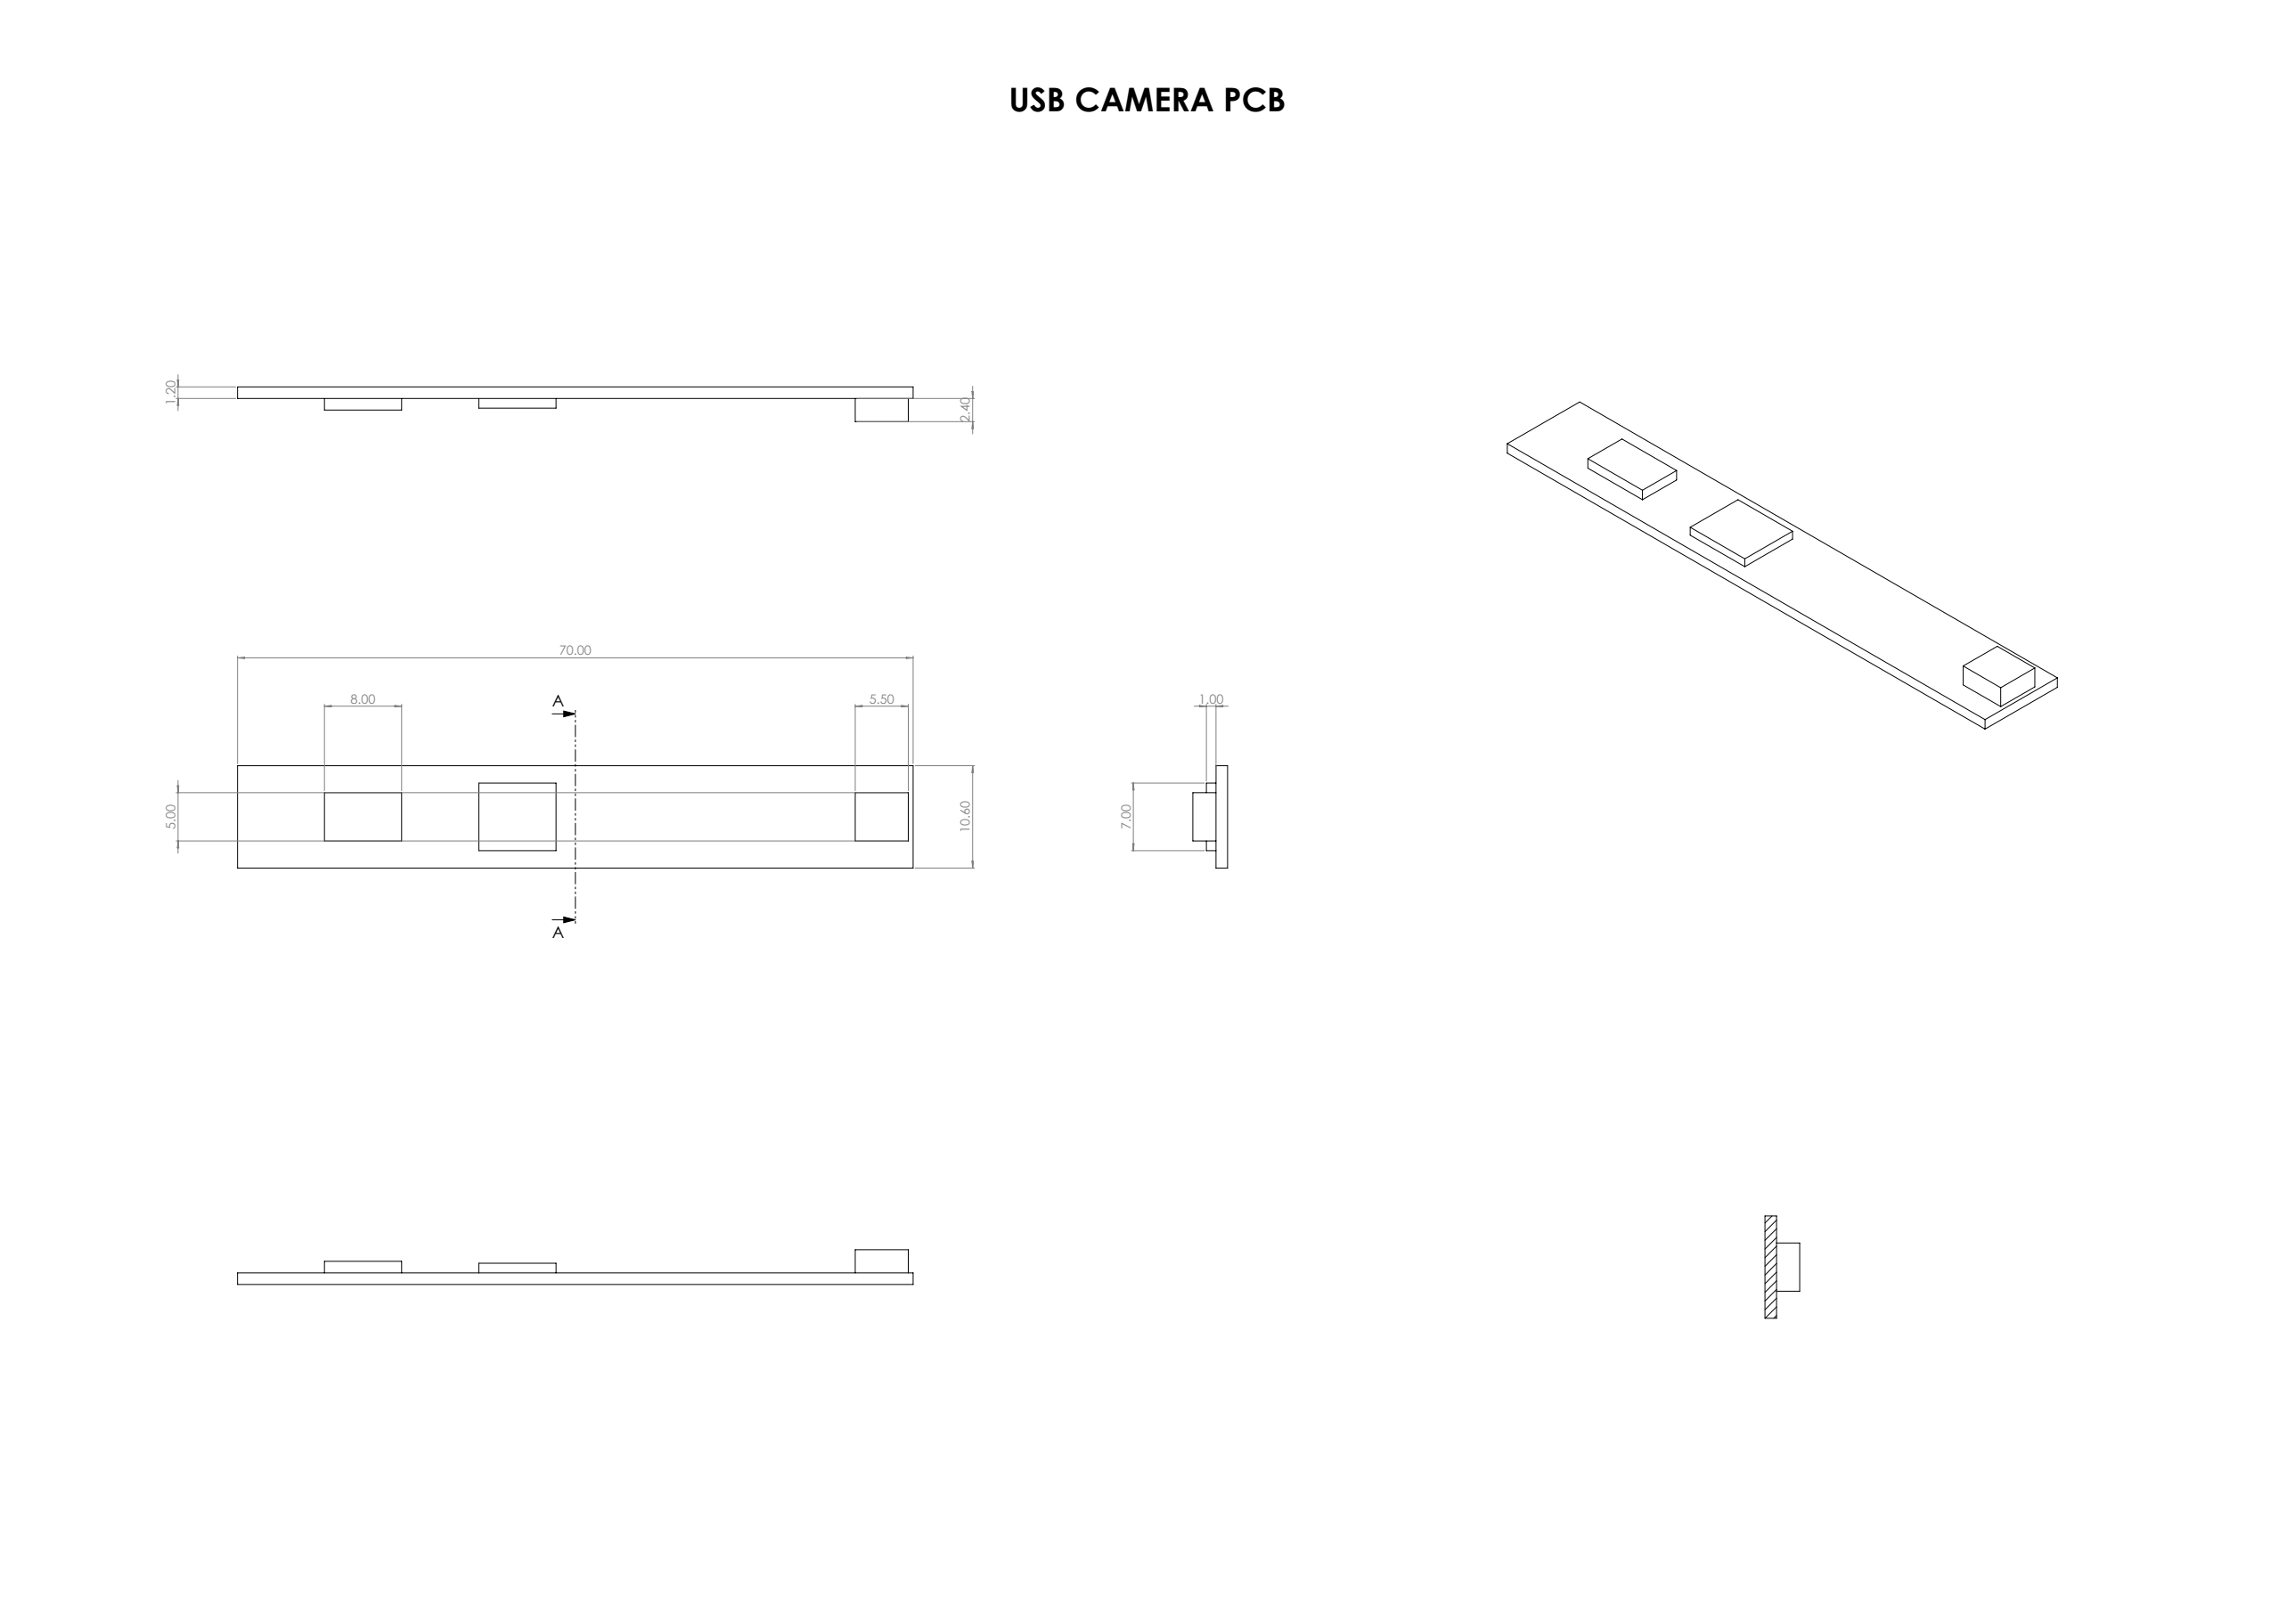
ISO-10303-21;
HEADER;
/* Generated by software containing ST-Developer
 * from STEP Tools, Inc. (www.steptools.com) 
 */

FILE_DESCRIPTION(
/* description */ (''),
/* implementation_level */ '2;1');

FILE_NAME(
/* name */ '05_USB_Camera_PCB.step',
/* time_stamp */ '2026-10-21T02:01:14-07:00',
/* author */ (''),
/* organization */ (''),
/* preprocessor_version */ 'ST-DEVELOPER v20.2',
/* originating_system */ 'Autodesk Translation Framework v15.15.0.0',
/* authorisation */ '');

FILE_SCHEMA (('AUTOMOTIVE_DESIGN { 1 0 10303 214 3 1 1 }'));
ENDSEC;

DATA;
#10=MECHANICAL_DESIGN_GEOMETRIC_PRESENTATION_REPRESENTATION('',(#618),#37181);
#592=SHAPE_REPRESENTATION_RELATIONSHIP('SRR','None',#37242,#605);
#605=ADVANCED_BREP_SHAPE_REPRESENTATION('',(#631),#37172);
#618=STYLED_ITEM('',(#37387),#631);
#631=MANIFOLD_SOLID_BREP('Body1',#14780);
#671=FACE_BOUND('',#2587,.T.);
#672=FACE_BOUND('',#2588,.T.);
#673=FACE_BOUND('',#2589,.T.);
#1696=FACE_OUTER_BOUND('',#2567,.T.);
#1697=FACE_OUTER_BOUND('',#2568,.T.);
#1698=FACE_OUTER_BOUND('',#2569,.T.);
#1699=FACE_OUTER_BOUND('',#2570,.T.);
#1700=FACE_OUTER_BOUND('',#2571,.T.);
#1701=FACE_OUTER_BOUND('',#2572,.T.);
#1702=FACE_OUTER_BOUND('',#2573,.T.);
#1703=FACE_OUTER_BOUND('',#2574,.T.);
#1704=FACE_OUTER_BOUND('',#2575,.T.);
#1705=FACE_OUTER_BOUND('',#2576,.T.);
#1706=FACE_OUTER_BOUND('',#2577,.T.);
#1707=FACE_OUTER_BOUND('',#2578,.T.);
#1708=FACE_OUTER_BOUND('',#2579,.T.);
#1709=FACE_OUTER_BOUND('',#2580,.T.);
#1710=FACE_OUTER_BOUND('',#2581,.T.);
#1711=FACE_OUTER_BOUND('',#2582,.T.);
#1712=FACE_OUTER_BOUND('',#2583,.T.);
#1713=FACE_OUTER_BOUND('',#2584,.T.);
#1714=FACE_OUTER_BOUND('',#2585,.T.);
#1715=FACE_OUTER_BOUND('',#2586,.T.);
#1716=FACE_OUTER_BOUND('',#2590,.T.);
#2567=EDGE_LOOP('',(#10741,#10742,#10743,#10744));
#2568=EDGE_LOOP('',(#10745,#10746,#10747,#10748));
#2569=EDGE_LOOP('',(#10749,#10750,#10751,#10752));
#2570=EDGE_LOOP('',(#10753,#10754,#10755,#10756));
#2571=EDGE_LOOP('',(#10757,#10758,#10759,#10760));
#2572=EDGE_LOOP('',(#10761,#10762,#10763,#10764));
#2573=EDGE_LOOP('',(#10765,#10766,#10767,#10768));
#2574=EDGE_LOOP('',(#10769,#10770,#10771,#10772));
#2575=EDGE_LOOP('',(#10773,#10774,#10775,#10776));
#2576=EDGE_LOOP('',(#10777,#10778,#10779,#10780));
#2577=EDGE_LOOP('',(#10781,#10782,#10783,#10784));
#2578=EDGE_LOOP('',(#10785,#10786,#10787,#10788));
#2579=EDGE_LOOP('',(#10789,#10790,#10791,#10792));
#2580=EDGE_LOOP('',(#10793,#10794,#10795,#10796));
#2581=EDGE_LOOP('',(#10797,#10798,#10799,#10800));
#2582=EDGE_LOOP('',(#10801,#10802,#10803,#10804));
#2583=EDGE_LOOP('',(#10805,#10806,#10807,#10808));
#2584=EDGE_LOOP('',(#10809,#10810,#10811,#10812));
#2585=EDGE_LOOP('',(#10813,#10814,#10815,#10816));
#2586=EDGE_LOOP('',(#10817,#10818,#10819,#10820));
#2587=EDGE_LOOP('',(#10821,#10822,#10823,#10824));
#2588=EDGE_LOOP('',(#10825,#10826,#10827,#10828));
#2589=EDGE_LOOP('',(#10829,#10830,#10831,#10832));
#2590=EDGE_LOOP('',(#10833,#10834,#10835,#10836));
#3784=LINE('',#21595,#5023);
#3785=LINE('',#21597,#5024);
#3786=LINE('',#21599,#5025);
#3787=LINE('',#21600,#5026);
#3788=LINE('',#21603,#5027);
#3789=LINE('',#21605,#5028);
#3790=LINE('',#21606,#5029);
#3791=LINE('',#21609,#5030);
#3792=LINE('',#21611,#5031);
#3793=LINE('',#21612,#5032);
#3794=LINE('',#21614,#5033);
#3795=LINE('',#21615,#5034);
#3796=LINE('',#21620,#5035);
#3797=LINE('',#21622,#5036);
#3798=LINE('',#21624,#5037);
#3799=LINE('',#21625,#5038);
#3800=LINE('',#21628,#5039);
#3801=LINE('',#21630,#5040);
#3802=LINE('',#21631,#5041);
#3803=LINE('',#21634,#5042);
#3804=LINE('',#21636,#5043);
#3805=LINE('',#21637,#5044);
#3806=LINE('',#21639,#5045);
#3807=LINE('',#21640,#5046);
#3808=LINE('',#21645,#5047);
#3809=LINE('',#21647,#5048);
#3810=LINE('',#21649,#5049);
#3811=LINE('',#21650,#5050);
#3812=LINE('',#21653,#5051);
#3813=LINE('',#21655,#5052);
#3814=LINE('',#21656,#5053);
#3815=LINE('',#21659,#5054);
#3816=LINE('',#21661,#5055);
#3817=LINE('',#21662,#5056);
#3818=LINE('',#21664,#5057);
#3819=LINE('',#21665,#5058);
#3820=LINE('',#21670,#5059);
#3821=LINE('',#21672,#5060);
#3822=LINE('',#21674,#5061);
#3823=LINE('',#21675,#5062);
#3824=LINE('',#21678,#5063);
#3825=LINE('',#21680,#5064);
#3826=LINE('',#21681,#5065);
#3827=LINE('',#21684,#5066);
#3828=LINE('',#21686,#5067);
#3829=LINE('',#21687,#5068);
#3830=LINE('',#21689,#5069);
#3831=LINE('',#21690,#5070);
#5023=VECTOR('',#17650,10.);
#5024=VECTOR('',#17651,10.);
#5025=VECTOR('',#17652,10.);
#5026=VECTOR('',#17653,10.);
#5027=VECTOR('',#17656,10.);
#5028=VECTOR('',#17657,10.);
#5029=VECTOR('',#17658,10.);
#5030=VECTOR('',#17661,10.);
#5031=VECTOR('',#17662,10.);
#5032=VECTOR('',#17663,10.);
#5033=VECTOR('',#17666,10.);
#5034=VECTOR('',#17667,10.);
#5035=VECTOR('',#17672,10.);
#5036=VECTOR('',#17673,10.);
#5037=VECTOR('',#17674,10.);
#5038=VECTOR('',#17675,10.);
#5039=VECTOR('',#17678,10.);
#5040=VECTOR('',#17679,10.);
#5041=VECTOR('',#17680,10.);
#5042=VECTOR('',#17683,10.);
#5043=VECTOR('',#17684,10.);
#5044=VECTOR('',#17685,10.);
#5045=VECTOR('',#17688,10.);
#5046=VECTOR('',#17689,10.);
#5047=VECTOR('',#17694,10.);
#5048=VECTOR('',#17695,10.);
#5049=VECTOR('',#17696,10.);
#5050=VECTOR('',#17697,10.);
#5051=VECTOR('',#17700,10.);
#5052=VECTOR('',#17701,10.);
#5053=VECTOR('',#17702,10.);
#5054=VECTOR('',#17705,10.);
#5055=VECTOR('',#17706,10.);
#5056=VECTOR('',#17707,10.);
#5057=VECTOR('',#17710,10.);
#5058=VECTOR('',#17711,10.);
#5059=VECTOR('',#17716,10.);
#5060=VECTOR('',#17717,10.);
#5061=VECTOR('',#17718,10.);
#5062=VECTOR('',#17719,10.);
#5063=VECTOR('',#17722,10.);
#5064=VECTOR('',#17723,10.);
#5065=VECTOR('',#17724,10.);
#5066=VECTOR('',#17727,10.);
#5067=VECTOR('',#17728,10.);
#5068=VECTOR('',#17729,10.);
#5069=VECTOR('',#17732,10.);
#5070=VECTOR('',#17733,10.);
#6151=VERTEX_POINT('',#21593);
#6152=VERTEX_POINT('',#21594);
#6153=VERTEX_POINT('',#21596);
#6154=VERTEX_POINT('',#21598);
#6155=VERTEX_POINT('',#21602);
#6156=VERTEX_POINT('',#21604);
#6157=VERTEX_POINT('',#21608);
#6158=VERTEX_POINT('',#21610);
#6159=VERTEX_POINT('',#21618);
#6160=VERTEX_POINT('',#21619);
#6161=VERTEX_POINT('',#21621);
#6162=VERTEX_POINT('',#21623);
#6163=VERTEX_POINT('',#21627);
#6164=VERTEX_POINT('',#21629);
#6165=VERTEX_POINT('',#21633);
#6166=VERTEX_POINT('',#21635);
#6167=VERTEX_POINT('',#21643);
#6168=VERTEX_POINT('',#21644);
#6169=VERTEX_POINT('',#21646);
#6170=VERTEX_POINT('',#21648);
#6171=VERTEX_POINT('',#21652);
#6172=VERTEX_POINT('',#21654);
#6173=VERTEX_POINT('',#21658);
#6174=VERTEX_POINT('',#21660);
#6175=VERTEX_POINT('',#21668);
#6176=VERTEX_POINT('',#21669);
#6177=VERTEX_POINT('',#21671);
#6178=VERTEX_POINT('',#21673);
#6179=VERTEX_POINT('',#21677);
#6180=VERTEX_POINT('',#21679);
#6181=VERTEX_POINT('',#21683);
#6182=VERTEX_POINT('',#21685);
#7812=EDGE_CURVE('',#6151,#6152,#3784,.T.);
#7813=EDGE_CURVE('',#6151,#6153,#3785,.T.);
#7814=EDGE_CURVE('',#6154,#6153,#3786,.T.);
#7815=EDGE_CURVE('',#6152,#6154,#3787,.T.);
#7816=EDGE_CURVE('',#6152,#6155,#3788,.T.);
#7817=EDGE_CURVE('',#6156,#6154,#3789,.T.);
#7818=EDGE_CURVE('',#6155,#6156,#3790,.T.);
#7819=EDGE_CURVE('',#6155,#6157,#3791,.T.);
#7820=EDGE_CURVE('',#6158,#6156,#3792,.T.);
#7821=EDGE_CURVE('',#6157,#6158,#3793,.T.);
#7822=EDGE_CURVE('',#6157,#6151,#3794,.T.);
#7823=EDGE_CURVE('',#6153,#6158,#3795,.T.);
#7824=EDGE_CURVE('',#6159,#6160,#3796,.T.);
#7825=EDGE_CURVE('',#6159,#6161,#3797,.T.);
#7826=EDGE_CURVE('',#6162,#6161,#3798,.T.);
#7827=EDGE_CURVE('',#6160,#6162,#3799,.T.);
#7828=EDGE_CURVE('',#6160,#6163,#3800,.T.);
#7829=EDGE_CURVE('',#6164,#6162,#3801,.T.);
#7830=EDGE_CURVE('',#6163,#6164,#3802,.T.);
#7831=EDGE_CURVE('',#6163,#6165,#3803,.T.);
#7832=EDGE_CURVE('',#6166,#6164,#3804,.T.);
#7833=EDGE_CURVE('',#6165,#6166,#3805,.T.);
#7834=EDGE_CURVE('',#6165,#6159,#3806,.T.);
#7835=EDGE_CURVE('',#6161,#6166,#3807,.T.);
#7836=EDGE_CURVE('',#6167,#6168,#3808,.T.);
#7837=EDGE_CURVE('',#6167,#6169,#3809,.T.);
#7838=EDGE_CURVE('',#6170,#6169,#3810,.T.);
#7839=EDGE_CURVE('',#6168,#6170,#3811,.T.);
#7840=EDGE_CURVE('',#6168,#6171,#3812,.T.);
#7841=EDGE_CURVE('',#6172,#6170,#3813,.T.);
#7842=EDGE_CURVE('',#6171,#6172,#3814,.T.);
#7843=EDGE_CURVE('',#6171,#6173,#3815,.T.);
#7844=EDGE_CURVE('',#6174,#6172,#3816,.T.);
#7845=EDGE_CURVE('',#6173,#6174,#3817,.T.);
#7846=EDGE_CURVE('',#6173,#6167,#3818,.T.);
#7847=EDGE_CURVE('',#6169,#6174,#3819,.T.);
#7848=EDGE_CURVE('',#6175,#6176,#3820,.T.);
#7849=EDGE_CURVE('',#6175,#6177,#3821,.T.);
#7850=EDGE_CURVE('',#6178,#6177,#3822,.T.);
#7851=EDGE_CURVE('',#6176,#6178,#3823,.T.);
#7852=EDGE_CURVE('',#6176,#6179,#3824,.T.);
#7853=EDGE_CURVE('',#6180,#6178,#3825,.T.);
#7854=EDGE_CURVE('',#6179,#6180,#3826,.T.);
#7855=EDGE_CURVE('',#6179,#6181,#3827,.T.);
#7856=EDGE_CURVE('',#6182,#6180,#3828,.T.);
#7857=EDGE_CURVE('',#6181,#6182,#3829,.T.);
#7858=EDGE_CURVE('',#6181,#6175,#3830,.T.);
#7859=EDGE_CURVE('',#6177,#6182,#3831,.T.);
#10741=ORIENTED_EDGE('',*,*,#7812,.F.);
#10742=ORIENTED_EDGE('',*,*,#7813,.T.);
#10743=ORIENTED_EDGE('',*,*,#7814,.F.);
#10744=ORIENTED_EDGE('',*,*,#7815,.F.);
#10745=ORIENTED_EDGE('',*,*,#7816,.F.);
#10746=ORIENTED_EDGE('',*,*,#7815,.T.);
#10747=ORIENTED_EDGE('',*,*,#7817,.F.);
#10748=ORIENTED_EDGE('',*,*,#7818,.F.);
#10749=ORIENTED_EDGE('',*,*,#7819,.F.);
#10750=ORIENTED_EDGE('',*,*,#7818,.T.);
#10751=ORIENTED_EDGE('',*,*,#7820,.F.);
#10752=ORIENTED_EDGE('',*,*,#7821,.F.);
#10753=ORIENTED_EDGE('',*,*,#7822,.F.);
#10754=ORIENTED_EDGE('',*,*,#7821,.T.);
#10755=ORIENTED_EDGE('',*,*,#7823,.F.);
#10756=ORIENTED_EDGE('',*,*,#7813,.F.);
#10757=ORIENTED_EDGE('',*,*,#7823,.T.);
#10758=ORIENTED_EDGE('',*,*,#7820,.T.);
#10759=ORIENTED_EDGE('',*,*,#7817,.T.);
#10760=ORIENTED_EDGE('',*,*,#7814,.T.);
#10761=ORIENTED_EDGE('',*,*,#7824,.F.);
#10762=ORIENTED_EDGE('',*,*,#7825,.T.);
#10763=ORIENTED_EDGE('',*,*,#7826,.F.);
#10764=ORIENTED_EDGE('',*,*,#7827,.F.);
#10765=ORIENTED_EDGE('',*,*,#7828,.F.);
#10766=ORIENTED_EDGE('',*,*,#7827,.T.);
#10767=ORIENTED_EDGE('',*,*,#7829,.F.);
#10768=ORIENTED_EDGE('',*,*,#7830,.F.);
#10769=ORIENTED_EDGE('',*,*,#7831,.F.);
#10770=ORIENTED_EDGE('',*,*,#7830,.T.);
#10771=ORIENTED_EDGE('',*,*,#7832,.F.);
#10772=ORIENTED_EDGE('',*,*,#7833,.F.);
#10773=ORIENTED_EDGE('',*,*,#7834,.F.);
#10774=ORIENTED_EDGE('',*,*,#7833,.T.);
#10775=ORIENTED_EDGE('',*,*,#7835,.F.);
#10776=ORIENTED_EDGE('',*,*,#7825,.F.);
#10777=ORIENTED_EDGE('',*,*,#7835,.T.);
#10778=ORIENTED_EDGE('',*,*,#7832,.T.);
#10779=ORIENTED_EDGE('',*,*,#7829,.T.);
#10780=ORIENTED_EDGE('',*,*,#7826,.T.);
#10781=ORIENTED_EDGE('',*,*,#7836,.F.);
#10782=ORIENTED_EDGE('',*,*,#7837,.T.);
#10783=ORIENTED_EDGE('',*,*,#7838,.F.);
#10784=ORIENTED_EDGE('',*,*,#7839,.F.);
#10785=ORIENTED_EDGE('',*,*,#7840,.F.);
#10786=ORIENTED_EDGE('',*,*,#7839,.T.);
#10787=ORIENTED_EDGE('',*,*,#7841,.F.);
#10788=ORIENTED_EDGE('',*,*,#7842,.F.);
#10789=ORIENTED_EDGE('',*,*,#7843,.F.);
#10790=ORIENTED_EDGE('',*,*,#7842,.T.);
#10791=ORIENTED_EDGE('',*,*,#7844,.F.);
#10792=ORIENTED_EDGE('',*,*,#7845,.F.);
#10793=ORIENTED_EDGE('',*,*,#7846,.F.);
#10794=ORIENTED_EDGE('',*,*,#7845,.T.);
#10795=ORIENTED_EDGE('',*,*,#7847,.F.);
#10796=ORIENTED_EDGE('',*,*,#7837,.F.);
#10797=ORIENTED_EDGE('',*,*,#7847,.T.);
#10798=ORIENTED_EDGE('',*,*,#7844,.T.);
#10799=ORIENTED_EDGE('',*,*,#7841,.T.);
#10800=ORIENTED_EDGE('',*,*,#7838,.T.);
#10801=ORIENTED_EDGE('',*,*,#7848,.F.);
#10802=ORIENTED_EDGE('',*,*,#7849,.T.);
#10803=ORIENTED_EDGE('',*,*,#7850,.F.);
#10804=ORIENTED_EDGE('',*,*,#7851,.F.);
#10805=ORIENTED_EDGE('',*,*,#7852,.F.);
#10806=ORIENTED_EDGE('',*,*,#7851,.T.);
#10807=ORIENTED_EDGE('',*,*,#7853,.F.);
#10808=ORIENTED_EDGE('',*,*,#7854,.F.);
#10809=ORIENTED_EDGE('',*,*,#7855,.F.);
#10810=ORIENTED_EDGE('',*,*,#7854,.T.);
#10811=ORIENTED_EDGE('',*,*,#7856,.F.);
#10812=ORIENTED_EDGE('',*,*,#7857,.F.);
#10813=ORIENTED_EDGE('',*,*,#7858,.F.);
#10814=ORIENTED_EDGE('',*,*,#7857,.T.);
#10815=ORIENTED_EDGE('',*,*,#7859,.F.);
#10816=ORIENTED_EDGE('',*,*,#7849,.F.);
#10817=ORIENTED_EDGE('',*,*,#7859,.T.);
#10818=ORIENTED_EDGE('',*,*,#7856,.T.);
#10819=ORIENTED_EDGE('',*,*,#7853,.T.);
#10820=ORIENTED_EDGE('',*,*,#7850,.T.);
#10821=ORIENTED_EDGE('',*,*,#7812,.T.);
#10822=ORIENTED_EDGE('',*,*,#7816,.T.);
#10823=ORIENTED_EDGE('',*,*,#7819,.T.);
#10824=ORIENTED_EDGE('',*,*,#7822,.T.);
#10825=ORIENTED_EDGE('',*,*,#7824,.T.);
#10826=ORIENTED_EDGE('',*,*,#7828,.T.);
#10827=ORIENTED_EDGE('',*,*,#7831,.T.);
#10828=ORIENTED_EDGE('',*,*,#7834,.T.);
#10829=ORIENTED_EDGE('',*,*,#7836,.T.);
#10830=ORIENTED_EDGE('',*,*,#7840,.T.);
#10831=ORIENTED_EDGE('',*,*,#7843,.T.);
#10832=ORIENTED_EDGE('',*,*,#7846,.T.);
#10833=ORIENTED_EDGE('',*,*,#7858,.T.);
#10834=ORIENTED_EDGE('',*,*,#7848,.T.);
#10835=ORIENTED_EDGE('',*,*,#7852,.T.);
#10836=ORIENTED_EDGE('',*,*,#7855,.T.);
#13679=PLANE('',#15404);
#13680=PLANE('',#15405);
#13681=PLANE('',#15406);
#13682=PLANE('',#15407);
#13683=PLANE('',#15408);
#13684=PLANE('',#15409);
#13685=PLANE('',#15410);
#13686=PLANE('',#15411);
#13687=PLANE('',#15412);
#13688=PLANE('',#15413);
#13689=PLANE('',#15414);
#13690=PLANE('',#15415);
#13691=PLANE('',#15416);
#13692=PLANE('',#15417);
#13693=PLANE('',#15418);
#13694=PLANE('',#15419);
#13695=PLANE('',#15420);
#13696=PLANE('',#15421);
#13697=PLANE('',#15422);
#13698=PLANE('',#15423);
#13699=PLANE('',#15424);
#14264=ADVANCED_FACE('',(#1696),#13679,.T.);
#14265=ADVANCED_FACE('',(#1697),#13680,.T.);
#14266=ADVANCED_FACE('',(#1698),#13681,.T.);
#14267=ADVANCED_FACE('',(#1699),#13682,.T.);
#14268=ADVANCED_FACE('',(#1700),#13683,.T.);
#14269=ADVANCED_FACE('',(#1701),#13684,.T.);
#14270=ADVANCED_FACE('',(#1702),#13685,.T.);
#14271=ADVANCED_FACE('',(#1703),#13686,.T.);
#14272=ADVANCED_FACE('',(#1704),#13687,.T.);
#14273=ADVANCED_FACE('',(#1705),#13688,.T.);
#14274=ADVANCED_FACE('',(#1706),#13689,.T.);
#14275=ADVANCED_FACE('',(#1707),#13690,.T.);
#14276=ADVANCED_FACE('',(#1708),#13691,.T.);
#14277=ADVANCED_FACE('',(#1709),#13692,.T.);
#14278=ADVANCED_FACE('',(#1710),#13693,.T.);
#14279=ADVANCED_FACE('',(#1711),#13694,.T.);
#14280=ADVANCED_FACE('',(#1712),#13695,.T.);
#14281=ADVANCED_FACE('',(#1713),#13696,.T.);
#14282=ADVANCED_FACE('',(#1714),#13697,.T.);
#14283=ADVANCED_FACE('',(#1715,#671,#672,#673),#13698,.T.);
#14284=ADVANCED_FACE('',(#1716),#13699,.F.);
#14780=CLOSED_SHELL('',(#14264,#14265,#14266,#14267,#14268,#14269,#14270,
#14271,#14272,#14273,#14274,#14275,#14276,#14277,#14278,#14279,#14280,#14281,
#14282,#14283,#14284));
#15403=AXIS2_PLACEMENT_3D('',#21591,#17646,#17647);
#15404=AXIS2_PLACEMENT_3D('',#21592,#17648,#17649);
#15405=AXIS2_PLACEMENT_3D('',#21601,#17654,#17655);
#15406=AXIS2_PLACEMENT_3D('',#21607,#17659,#17660);
#15407=AXIS2_PLACEMENT_3D('',#21613,#17664,#17665);
#15408=AXIS2_PLACEMENT_3D('',#21616,#17668,#17669);
#15409=AXIS2_PLACEMENT_3D('',#21617,#17670,#17671);
#15410=AXIS2_PLACEMENT_3D('',#21626,#17676,#17677);
#15411=AXIS2_PLACEMENT_3D('',#21632,#17681,#17682);
#15412=AXIS2_PLACEMENT_3D('',#21638,#17686,#17687);
#15413=AXIS2_PLACEMENT_3D('',#21641,#17690,#17691);
#15414=AXIS2_PLACEMENT_3D('',#21642,#17692,#17693);
#15415=AXIS2_PLACEMENT_3D('',#21651,#17698,#17699);
#15416=AXIS2_PLACEMENT_3D('',#21657,#17703,#17704);
#15417=AXIS2_PLACEMENT_3D('',#21663,#17708,#17709);
#15418=AXIS2_PLACEMENT_3D('',#21666,#17712,#17713);
#15419=AXIS2_PLACEMENT_3D('',#21667,#17714,#17715);
#15420=AXIS2_PLACEMENT_3D('',#21676,#17720,#17721);
#15421=AXIS2_PLACEMENT_3D('',#21682,#17725,#17726);
#15422=AXIS2_PLACEMENT_3D('',#21688,#17730,#17731);
#15423=AXIS2_PLACEMENT_3D('',#21691,#17734,#17735);
#15424=AXIS2_PLACEMENT_3D('',#21692,#17736,#17737);
#17646=DIRECTION('axis',(0.,0.,1.));
#17647=DIRECTION('refdir',(1.,0.,0.));
#17648=DIRECTION('center_axis',(-1.,0.,0.));
#17649=DIRECTION('ref_axis',(0.,0.,1.));
#17650=DIRECTION('',(0.,0.,-1.));
#17651=DIRECTION('',(0.,1.,0.));
#17652=DIRECTION('',(0.,0.,1.));
#17653=DIRECTION('',(0.,1.,0.));
#17654=DIRECTION('center_axis',(0.,0.,-1.));
#17655=DIRECTION('ref_axis',(-1.,0.,0.));
#17656=DIRECTION('',(1.,0.,0.));
#17657=DIRECTION('',(-1.,0.,0.));
#17658=DIRECTION('',(0.,1.,0.));
#17659=DIRECTION('center_axis',(1.,0.,0.));
#17660=DIRECTION('ref_axis',(0.,0.,-1.));
#17661=DIRECTION('',(0.,0.,1.));
#17662=DIRECTION('',(0.,0.,-1.));
#17663=DIRECTION('',(0.,1.,0.));
#17664=DIRECTION('center_axis',(0.,0.,1.));
#17665=DIRECTION('ref_axis',(1.,0.,0.));
#17666=DIRECTION('',(-1.,0.,0.));
#17667=DIRECTION('',(1.,0.,0.));
#17668=DIRECTION('center_axis',(0.,1.,0.));
#17669=DIRECTION('ref_axis',(0.,0.,1.));
#17670=DIRECTION('center_axis',(-1.,0.,0.));
#17671=DIRECTION('ref_axis',(0.,0.,1.));
#17672=DIRECTION('',(0.,0.,-1.));
#17673=DIRECTION('',(0.,1.,0.));
#17674=DIRECTION('',(0.,0.,1.));
#17675=DIRECTION('',(0.,1.,0.));
#17676=DIRECTION('center_axis',(0.,0.,-1.));
#17677=DIRECTION('ref_axis',(-1.,0.,0.));
#17678=DIRECTION('',(1.,0.,0.));
#17679=DIRECTION('',(-1.,0.,0.));
#17680=DIRECTION('',(0.,1.,0.));
#17681=DIRECTION('center_axis',(1.,0.,0.));
#17682=DIRECTION('ref_axis',(0.,0.,-1.));
#17683=DIRECTION('',(0.,0.,1.));
#17684=DIRECTION('',(0.,0.,-1.));
#17685=DIRECTION('',(0.,1.,0.));
#17686=DIRECTION('center_axis',(0.,0.,1.));
#17687=DIRECTION('ref_axis',(1.,0.,0.));
#17688=DIRECTION('',(-1.,0.,0.));
#17689=DIRECTION('',(1.,0.,0.));
#17690=DIRECTION('center_axis',(0.,1.,0.));
#17691=DIRECTION('ref_axis',(0.,0.,1.));
#17692=DIRECTION('center_axis',(-1.,0.,0.));
#17693=DIRECTION('ref_axis',(0.,0.,1.));
#17694=DIRECTION('',(0.,0.,-1.));
#17695=DIRECTION('',(0.,1.,0.));
#17696=DIRECTION('',(0.,0.,1.));
#17697=DIRECTION('',(0.,1.,0.));
#17698=DIRECTION('center_axis',(0.,0.,-1.));
#17699=DIRECTION('ref_axis',(-1.,0.,0.));
#17700=DIRECTION('',(1.,0.,0.));
#17701=DIRECTION('',(-1.,0.,0.));
#17702=DIRECTION('',(0.,1.,0.));
#17703=DIRECTION('center_axis',(1.,0.,0.));
#17704=DIRECTION('ref_axis',(0.,0.,-1.));
#17705=DIRECTION('',(0.,0.,1.));
#17706=DIRECTION('',(0.,0.,-1.));
#17707=DIRECTION('',(0.,1.,0.));
#17708=DIRECTION('center_axis',(0.,0.,1.));
#17709=DIRECTION('ref_axis',(1.,0.,0.));
#17710=DIRECTION('',(-1.,0.,0.));
#17711=DIRECTION('',(1.,0.,0.));
#17712=DIRECTION('center_axis',(0.,1.,0.));
#17713=DIRECTION('ref_axis',(0.,0.,1.));
#17714=DIRECTION('center_axis',(-1.,0.,0.));
#17715=DIRECTION('ref_axis',(0.,0.,1.));
#17716=DIRECTION('',(0.,0.,-1.));
#17717=DIRECTION('',(0.,1.,0.));
#17718=DIRECTION('',(0.,0.,1.));
#17719=DIRECTION('',(0.,1.,0.));
#17720=DIRECTION('center_axis',(0.,0.,-1.));
#17721=DIRECTION('ref_axis',(-1.,0.,0.));
#17722=DIRECTION('',(1.,0.,0.));
#17723=DIRECTION('',(-1.,0.,0.));
#17724=DIRECTION('',(0.,1.,0.));
#17725=DIRECTION('center_axis',(1.,0.,0.));
#17726=DIRECTION('ref_axis',(0.,0.,-1.));
#17727=DIRECTION('',(0.,0.,1.));
#17728=DIRECTION('',(0.,0.,-1.));
#17729=DIRECTION('',(0.,1.,0.));
#17730=DIRECTION('center_axis',(0.,0.,1.));
#17731=DIRECTION('ref_axis',(1.,0.,0.));
#17732=DIRECTION('',(-1.,0.,0.));
#17733=DIRECTION('',(1.,0.,0.));
#17734=DIRECTION('center_axis',(0.,1.,0.));
#17735=DIRECTION('ref_axis',(0.,0.,1.));
#17736=DIRECTION('center_axis',(0.,1.,0.));
#17737=DIRECTION('ref_axis',(1.,0.,0.));
#21591=CARTESIAN_POINT('',(0.,0.,0.));
#21592=CARTESIAN_POINT('Origin',(-22.,-7.8,-50.));
#21593=CARTESIAN_POINT('',(-22.,-7.8,-45.));
#21594=CARTESIAN_POINT('',(-22.,-7.8,-50.));
#21595=CARTESIAN_POINT('',(-22.,-7.8,-48.75));
#21596=CARTESIAN_POINT('',(-22.,-6.6,-45.));
#21597=CARTESIAN_POINT('',(-22.,-7.8,-45.));
#21598=CARTESIAN_POINT('',(-22.,-6.6,-50.));
#21599=CARTESIAN_POINT('',(-22.,-6.6,-45.));
#21600=CARTESIAN_POINT('',(-22.,-7.8,-50.));
#21601=CARTESIAN_POINT('Origin',(-14.,-7.8,-50.));
#21602=CARTESIAN_POINT('',(-14.,-7.8,-50.));
#21603=CARTESIAN_POINT('',(-5.,-7.8,-50.));
#21604=CARTESIAN_POINT('',(-14.,-6.6,-50.));
#21605=CARTESIAN_POINT('',(-22.,-6.6,-50.));
#21606=CARTESIAN_POINT('',(-14.,-7.8,-50.));
#21607=CARTESIAN_POINT('Origin',(-14.,-7.8,-45.));
#21608=CARTESIAN_POINT('',(-14.,-7.8,-45.));
#21609=CARTESIAN_POINT('',(-14.,-7.8,-46.25));
#21610=CARTESIAN_POINT('',(-14.,-6.6,-45.));
#21611=CARTESIAN_POINT('',(-14.,-6.6,-50.));
#21612=CARTESIAN_POINT('',(-14.,-7.8,-45.));
#21613=CARTESIAN_POINT('Origin',(-22.,-7.8,-45.));
#21614=CARTESIAN_POINT('',(-9.,-7.8,-45.));
#21615=CARTESIAN_POINT('',(-14.,-6.6,-45.));
#21616=CARTESIAN_POINT('Origin',(-18.,-6.6,-47.5));
#21617=CARTESIAN_POINT('Origin',(-6.,-7.8,-51.));
#21618=CARTESIAN_POINT('',(-6.,-7.8,-44.));
#21619=CARTESIAN_POINT('',(-6.,-7.8,-51.));
#21620=CARTESIAN_POINT('',(-6.,-7.8,-49.25));
#21621=CARTESIAN_POINT('',(-6.,-6.8,-44.));
#21622=CARTESIAN_POINT('',(-6.,-7.8,-44.));
#21623=CARTESIAN_POINT('',(-6.,-6.8,-51.));
#21624=CARTESIAN_POINT('',(-6.,-6.8,-44.));
#21625=CARTESIAN_POINT('',(-6.,-7.8,-51.));
#21626=CARTESIAN_POINT('Origin',(2.,-7.8,-51.));
#21627=CARTESIAN_POINT('',(2.,-7.8,-51.));
#21628=CARTESIAN_POINT('',(3.,-7.8,-51.));
#21629=CARTESIAN_POINT('',(2.,-6.8,-51.));
#21630=CARTESIAN_POINT('',(-6.,-6.8,-51.));
#21631=CARTESIAN_POINT('',(2.,-7.8,-51.));
#21632=CARTESIAN_POINT('Origin',(2.,-7.8,-44.));
#21633=CARTESIAN_POINT('',(2.,-7.8,-44.));
#21634=CARTESIAN_POINT('',(2.,-7.8,-45.75));
#21635=CARTESIAN_POINT('',(2.,-6.8,-44.));
#21636=CARTESIAN_POINT('',(2.,-6.8,-51.));
#21637=CARTESIAN_POINT('',(2.,-7.8,-44.));
#21638=CARTESIAN_POINT('Origin',(-6.,-7.8,-44.));
#21639=CARTESIAN_POINT('',(-1.,-7.8,-44.));
#21640=CARTESIAN_POINT('',(2.,-6.8,-44.));
#21641=CARTESIAN_POINT('Origin',(-2.,-6.8,-47.5));
#21642=CARTESIAN_POINT('Origin',(33.,-7.8,-50.));
#21643=CARTESIAN_POINT('',(33.,-7.8,-45.));
#21644=CARTESIAN_POINT('',(33.,-7.8,-50.));
#21645=CARTESIAN_POINT('',(33.,-7.8,-48.75));
#21646=CARTESIAN_POINT('',(33.,-5.4,-45.));
#21647=CARTESIAN_POINT('',(33.,-7.8,-45.));
#21648=CARTESIAN_POINT('',(33.,-5.4,-50.));
#21649=CARTESIAN_POINT('',(33.,-5.4,-45.));
#21650=CARTESIAN_POINT('',(33.,-7.8,-50.));
#21651=CARTESIAN_POINT('Origin',(38.5,-7.8,-50.));
#21652=CARTESIAN_POINT('',(38.5,-7.8,-50.));
#21653=CARTESIAN_POINT('',(21.25,-7.8,-50.));
#21654=CARTESIAN_POINT('',(38.5,-5.4,-50.));
#21655=CARTESIAN_POINT('',(33.,-5.4,-50.));
#21656=CARTESIAN_POINT('',(38.5,-7.8,-50.));
#21657=CARTESIAN_POINT('Origin',(38.5,-7.8,-45.));
#21658=CARTESIAN_POINT('',(38.5,-7.8,-45.));
#21659=CARTESIAN_POINT('',(38.5,-7.8,-46.25));
#21660=CARTESIAN_POINT('',(38.5,-5.4,-45.));
#21661=CARTESIAN_POINT('',(38.5,-5.4,-50.));
#21662=CARTESIAN_POINT('',(38.5,-7.8,-45.));
#21663=CARTESIAN_POINT('Origin',(33.,-7.8,-45.));
#21664=CARTESIAN_POINT('',(18.5,-7.8,-45.));
#21665=CARTESIAN_POINT('',(38.5,-5.4,-45.));
#21666=CARTESIAN_POINT('Origin',(35.75,-5.4,-47.5));
#21667=CARTESIAN_POINT('Origin',(-31.,-9.,-52.8));
#21668=CARTESIAN_POINT('',(-31.,-9.,-42.2));
#21669=CARTESIAN_POINT('',(-31.,-9.,-52.8));
#21670=CARTESIAN_POINT('',(-31.,-9.,-42.2));
#21671=CARTESIAN_POINT('',(-31.,-7.8,-42.2));
#21672=CARTESIAN_POINT('',(-31.,-9.,-42.2));
#21673=CARTESIAN_POINT('',(-31.,-7.8,-52.8));
#21674=CARTESIAN_POINT('',(-31.,-7.8,-42.2));
#21675=CARTESIAN_POINT('',(-31.,-9.,-52.8));
#21676=CARTESIAN_POINT('Origin',(39.,-9.,-52.8));
#21677=CARTESIAN_POINT('',(39.,-9.,-52.8));
#21678=CARTESIAN_POINT('',(-31.,-9.,-52.8));
#21679=CARTESIAN_POINT('',(39.,-7.8,-52.8));
#21680=CARTESIAN_POINT('',(-31.,-7.8,-52.8));
#21681=CARTESIAN_POINT('',(39.,-9.,-52.8));
#21682=CARTESIAN_POINT('Origin',(39.,-9.,-42.2));
#21683=CARTESIAN_POINT('',(39.,-9.,-42.2));
#21684=CARTESIAN_POINT('',(39.,-9.,-52.8));
#21685=CARTESIAN_POINT('',(39.,-7.8,-42.2));
#21686=CARTESIAN_POINT('',(39.,-7.8,-52.8));
#21687=CARTESIAN_POINT('',(39.,-9.,-42.2));
#21688=CARTESIAN_POINT('Origin',(-31.,-9.,-42.2));
#21689=CARTESIAN_POINT('',(39.,-9.,-42.2));
#21690=CARTESIAN_POINT('',(39.,-7.8,-42.2));
#21691=CARTESIAN_POINT('Origin',(4.,-7.8,-47.5));
#21692=CARTESIAN_POINT('Origin',(4.,-9.,-47.5));
#37157=UNCERTAINTY_MEASURE_WITH_UNIT(LENGTH_MEASURE(0.01),#37182,
'DISTANCE_ACCURACY_VALUE',
'Maximum model space distance between geometric entities at asserted c
onnectivities');
#37166=UNCERTAINTY_MEASURE_WITH_UNIT(LENGTH_MEASURE(0.01),#37182,
'DISTANCE_ACCURACY_VALUE',
'Maximum model space distance between geometric entities at asserted c
onnectivities');
#37172=(
GEOMETRIC_REPRESENTATION_CONTEXT(3)
GLOBAL_UNCERTAINTY_ASSIGNED_CONTEXT((#37157))
GLOBAL_UNIT_ASSIGNED_CONTEXT((#37182,#37184,#37185))
REPRESENTATION_CONTEXT('','3D')
);
#37181=(
GEOMETRIC_REPRESENTATION_CONTEXT(3)
GLOBAL_UNCERTAINTY_ASSIGNED_CONTEXT((#37166))
GLOBAL_UNIT_ASSIGNED_CONTEXT((#37182,#37184,#37185))
REPRESENTATION_CONTEXT('','3D')
);
#37182=(
LENGTH_UNIT()
NAMED_UNIT(*)
SI_UNIT(.MILLI.,.METRE.)
);
#37184=(
NAMED_UNIT(*)
PLANE_ANGLE_UNIT()
SI_UNIT($,.RADIAN.)
);
#37185=(
NAMED_UNIT(*)
SI_UNIT($,.STERADIAN.)
SOLID_ANGLE_UNIT()
);
#37191=SHAPE_DEFINITION_REPRESENTATION(#37205,#37242);
#37205=PRODUCT_DEFINITION_SHAPE('',$,#37257);
#37242=SHAPE_REPRESENTATION('',(#15403),#37172);
#37251=PRODUCT_DEFINITION_CONTEXT('part definition',#37295,'design');
#37257=PRODUCT_DEFINITION('2026-10-20-13-23-54-211','05_USB_Camera_PCB',
#37271,#37251);
#37271=PRODUCT_DEFINITION_FORMATION('',$,#37302);
#37295=APPLICATION_CONTEXT(
'Core Data for Automotive Mechanical Design Process');
#37296=PRODUCT_CONTEXT('part definition',#37295,'mechanical');
#37302=PRODUCT('2026-10-20-13-23-54-211','05_USB_Camera_PCB',$,(#37296));
#37381=COLOUR_RGB('Off White',0.89,0.88,0.83);
#37382=FILL_AREA_STYLE_COLOUR('',#37381);
#37383=FILL_AREA_STYLE('',(#37382));
#37384=SURFACE_STYLE_FILL_AREA(#37383);
#37385=SURFACE_SIDE_STYLE('',(#37384));
#37386=SURFACE_STYLE_USAGE(.BOTH.,#37385);
#37387=PRESENTATION_STYLE_ASSIGNMENT((#37386));
ENDSEC;
END-ISO-10303-21;
